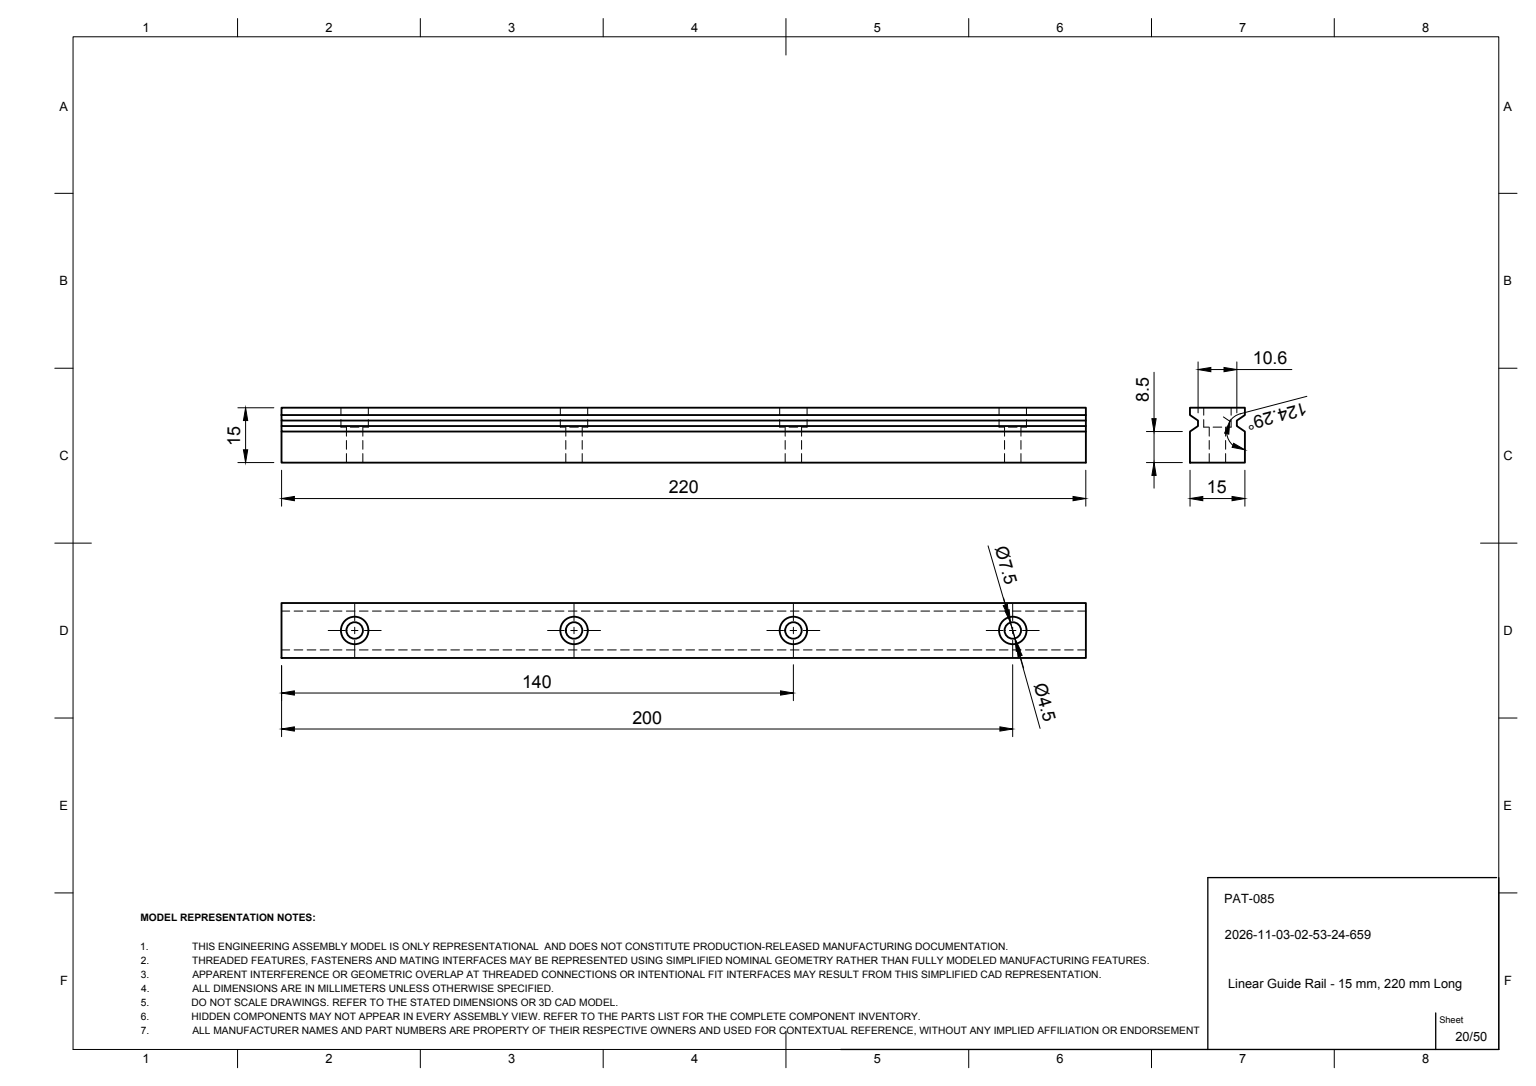
ISO-10303-21;
HEADER;
/* Generated by software containing ST-Developer
 * from STEP Tools, Inc. (www.steptools.com) 
 */

FILE_DESCRIPTION(
/* description */ ('Rack and pinion manual slide'),
/* implementation_level */ '2;1');

FILE_NAME(
/* name */ 'Linear Guide Rail - 15 mm, 220 mm Long.step',
/* time_stamp */ '2026-10-28T03:22:49-07:00',
/* author */ (''),
/* organization */ (''),
/* preprocessor_version */ 'ST-DEVELOPER v20.2',
/* originating_system */ 'Autodesk Translation Framework v15.17.0.0',
/* authorisation */ '');

FILE_SCHEMA (('AUTOMOTIVE_DESIGN { 1 0 10303 214 3 1 1 }'));
ENDSEC;

DATA;
#10=MECHANICAL_DESIGN_GEOMETRIC_PRESENTATION_REPRESENTATION('',(#749),#34851);
#657=SHAPE_REPRESENTATION_RELATIONSHIP('SRR','None',#35092,#703);
#703=ADVANCED_BREP_SHAPE_REPRESENTATION('',(#802),#34817);
#749=STYLED_ITEM('',(#35404),#802);
#802=MANIFOLD_SOLID_BREP('Body1',#13769);
#962=FACE_BOUND('',#2625,.T.);
#963=FACE_BOUND('',#2628,.T.);
#964=FACE_BOUND('',#2631,.T.);
#965=FACE_BOUND('',#2634,.T.);
#966=FACE_BOUND('',#2644,.T.);
#967=FACE_BOUND('',#2645,.T.);
#968=FACE_BOUND('',#2646,.T.);
#969=FACE_BOUND('',#2647,.T.);
#970=FACE_BOUND('',#2654,.T.);
#971=FACE_BOUND('',#2655,.T.);
#972=FACE_BOUND('',#2656,.T.);
#973=FACE_BOUND('',#2657,.T.);
#1189=PLANE('',#14713);
#1190=PLANE('',#14718);
#1191=PLANE('',#14723);
#1192=PLANE('',#14728);
#1193=PLANE('',#14738);
#1194=PLANE('',#14739);
#1195=PLANE('',#14740);
#1196=PLANE('',#14741);
#1197=PLANE('',#14742);
#1198=PLANE('',#14743);
#1199=PLANE('',#14744);
#1200=PLANE('',#14745);
#1201=PLANE('',#14746);
#1202=PLANE('',#14747);
#1203=PLANE('',#14748);
#1204=PLANE('',#14749);
#1205=PLANE('',#14750);
#1206=PLANE('',#14751);
#1755=FACE_OUTER_BOUND('',#2623,.T.);
#1756=FACE_OUTER_BOUND('',#2624,.T.);
#1757=FACE_OUTER_BOUND('',#2626,.T.);
#1758=FACE_OUTER_BOUND('',#2627,.T.);
#1759=FACE_OUTER_BOUND('',#2629,.T.);
#1760=FACE_OUTER_BOUND('',#2630,.T.);
#1761=FACE_OUTER_BOUND('',#2632,.T.);
#1762=FACE_OUTER_BOUND('',#2633,.T.);
#1763=FACE_OUTER_BOUND('',#2635,.T.);
#1764=FACE_OUTER_BOUND('',#2636,.T.);
#1765=FACE_OUTER_BOUND('',#2637,.T.);
#1766=FACE_OUTER_BOUND('',#2638,.T.);
#1767=FACE_OUTER_BOUND('',#2639,.T.);
#1768=FACE_OUTER_BOUND('',#2640,.T.);
#1769=FACE_OUTER_BOUND('',#2641,.T.);
#1770=FACE_OUTER_BOUND('',#2642,.T.);
#1771=FACE_OUTER_BOUND('',#2643,.T.);
#1772=FACE_OUTER_BOUND('',#2648,.T.);
#1773=FACE_OUTER_BOUND('',#2649,.T.);
#1774=FACE_OUTER_BOUND('',#2650,.T.);
#1775=FACE_OUTER_BOUND('',#2651,.T.);
#1776=FACE_OUTER_BOUND('',#2652,.T.);
#1777=FACE_OUTER_BOUND('',#2653,.T.);
#1778=FACE_OUTER_BOUND('',#2658,.T.);
#1779=FACE_OUTER_BOUND('',#2659,.T.);
#1780=FACE_OUTER_BOUND('',#2660,.T.);
#2623=EDGE_LOOP('',(#10306,#10307,#10308,#10309));
#2624=EDGE_LOOP('',(#10310));
#2625=EDGE_LOOP('',(#10311));
#2626=EDGE_LOOP('',(#10312,#10313,#10314,#10315));
#2627=EDGE_LOOP('',(#10316));
#2628=EDGE_LOOP('',(#10317));
#2629=EDGE_LOOP('',(#10318,#10319,#10320,#10321));
#2630=EDGE_LOOP('',(#10322));
#2631=EDGE_LOOP('',(#10323));
#2632=EDGE_LOOP('',(#10324,#10325,#10326,#10327));
#2633=EDGE_LOOP('',(#10328));
#2634=EDGE_LOOP('',(#10329));
#2635=EDGE_LOOP('',(#10330,#10331,#10332,#10333));
#2636=EDGE_LOOP('',(#10334,#10335,#10336,#10337));
#2637=EDGE_LOOP('',(#10338,#10339,#10340,#10341));
#2638=EDGE_LOOP('',(#10342,#10343,#10344,#10345));
#2639=EDGE_LOOP('',(#10346,#10347,#10348,#10349));
#2640=EDGE_LOOP('',(#10350,#10351,#10352,#10353));
#2641=EDGE_LOOP('',(#10354,#10355,#10356,#10357));
#2642=EDGE_LOOP('',(#10358,#10359,#10360,#10361));
#2643=EDGE_LOOP('',(#10362,#10363,#10364,#10365));
#2644=EDGE_LOOP('',(#10366));
#2645=EDGE_LOOP('',(#10367));
#2646=EDGE_LOOP('',(#10368));
#2647=EDGE_LOOP('',(#10369));
#2648=EDGE_LOOP('',(#10370,#10371,#10372,#10373));
#2649=EDGE_LOOP('',(#10374,#10375,#10376,#10377));
#2650=EDGE_LOOP('',(#10378,#10379,#10380,#10381));
#2651=EDGE_LOOP('',(#10382,#10383,#10384,#10385));
#2652=EDGE_LOOP('',(#10386,#10387,#10388,#10389));
#2653=EDGE_LOOP('',(#10390,#10391,#10392,#10393));
#2654=EDGE_LOOP('',(#10394));
#2655=EDGE_LOOP('',(#10395));
#2656=EDGE_LOOP('',(#10396));
#2657=EDGE_LOOP('',(#10397));
#2658=EDGE_LOOP('',(#10398,#10399,#10400,#10401));
#2659=EDGE_LOOP('',(#10402,#10403,#10404,#10405,#10406,#10407,#10408,#10409,
#10410,#10411,#10412,#10413));
#2660=EDGE_LOOP('',(#10414,#10415,#10416,#10417,#10418,#10419,#10420,#10421,
#10422,#10423,#10424,#10425));
#3607=LINE('',#20594,#4898);
#3608=LINE('',#20603,#4899);
#3609=LINE('',#20612,#4900);
#3610=LINE('',#20621,#4901);
#3611=LINE('',#20629,#4902);
#3612=LINE('',#20633,#4903);
#3613=LINE('',#20637,#4904);
#3614=LINE('',#20641,#4905);
#3615=LINE('',#20645,#4906);
#3616=LINE('',#20647,#4907);
#3617=LINE('',#20649,#4908);
#3618=LINE('',#20650,#4909);
#3619=LINE('',#20653,#4910);
#3620=LINE('',#20655,#4911);
#3621=LINE('',#20656,#4912);
#3622=LINE('',#20659,#4913);
#3623=LINE('',#20661,#4914);
#3624=LINE('',#20662,#4915);
#3625=LINE('',#20665,#4916);
#3626=LINE('',#20667,#4917);
#3627=LINE('',#20668,#4918);
#3628=LINE('',#20671,#4919);
#3629=LINE('',#20673,#4920);
#3630=LINE('',#20674,#4921);
#3631=LINE('',#20677,#4922);
#3632=LINE('',#20679,#4923);
#3633=LINE('',#20680,#4924);
#3634=LINE('',#20683,#4925);
#3635=LINE('',#20685,#4926);
#3636=LINE('',#20686,#4927);
#3637=LINE('',#20689,#4928);
#3638=LINE('',#20691,#4929);
#3639=LINE('',#20692,#4930);
#3640=LINE('',#20695,#4931);
#3641=LINE('',#20697,#4932);
#3642=LINE('',#20698,#4933);
#3643=LINE('',#20701,#4934);
#3644=LINE('',#20703,#4935);
#3645=LINE('',#20704,#4936);
#3646=LINE('',#20707,#4937);
#3647=LINE('',#20709,#4938);
#3648=LINE('',#20710,#4939);
#3649=LINE('',#20712,#4940);
#3650=LINE('',#20713,#4941);
#4898=VECTOR('',#16773,0.375);
#4899=VECTOR('',#16784,0.375);
#4900=VECTOR('',#16795,0.375);
#4901=VECTOR('',#16806,0.375);
#4902=VECTOR('',#16817,0.225);
#4903=VECTOR('',#16822,0.225);
#4904=VECTOR('',#16827,0.225);
#4905=VECTOR('',#16832,0.225000000000001);
#4906=VECTOR('',#16835,1.);
#4907=VECTOR('',#16836,1.);
#4908=VECTOR('',#16837,1.);
#4909=VECTOR('',#16838,1.);
#4910=VECTOR('',#16841,1.);
#4911=VECTOR('',#16842,1.);
#4912=VECTOR('',#16843,1.);
#4913=VECTOR('',#16846,1.);
#4914=VECTOR('',#16847,1.);
#4915=VECTOR('',#16848,1.);
#4916=VECTOR('',#16851,1.);
#4917=VECTOR('',#16852,1.);
#4918=VECTOR('',#16853,1.);
#4919=VECTOR('',#16856,1.);
#4920=VECTOR('',#16857,1.);
#4921=VECTOR('',#16858,1.);
#4922=VECTOR('',#16861,1.);
#4923=VECTOR('',#16862,1.);
#4924=VECTOR('',#16863,1.);
#4925=VECTOR('',#16866,1.);
#4926=VECTOR('',#16867,1.);
#4927=VECTOR('',#16868,1.);
#4928=VECTOR('',#16871,1.);
#4929=VECTOR('',#16872,1.);
#4930=VECTOR('',#16873,1.);
#4931=VECTOR('',#16876,1.);
#4932=VECTOR('',#16877,1.);
#4933=VECTOR('',#16878,1.);
#4934=VECTOR('',#16881,1.);
#4935=VECTOR('',#16882,1.);
#4936=VECTOR('',#16883,1.);
#4937=VECTOR('',#16886,1.);
#4938=VECTOR('',#16887,1.);
#4939=VECTOR('',#16888,1.);
#4940=VECTOR('',#16891,1.);
#4941=VECTOR('',#16892,1.);
#5957=CIRCLE('',#14711,0.375);
#5958=CIRCLE('',#14712,0.375);
#5959=CIRCLE('',#14714,0.225);
#5960=CIRCLE('',#14716,0.375);
#5961=CIRCLE('',#14717,0.375);
#5962=CIRCLE('',#14719,0.225);
#5963=CIRCLE('',#14721,0.375);
#5964=CIRCLE('',#14722,0.375);
#5965=CIRCLE('',#14724,0.225);
#5966=CIRCLE('',#14726,0.375);
#5967=CIRCLE('',#14727,0.375);
#5968=CIRCLE('',#14729,0.225000000000001);
#5969=CIRCLE('',#14731,0.225);
#5970=CIRCLE('',#14733,0.225);
#5971=CIRCLE('',#14735,0.225);
#5972=CIRCLE('',#14737,0.225000000000001);
#6581=VERTEX_POINT('',#20591);
#6582=VERTEX_POINT('',#20593);
#6583=VERTEX_POINT('',#20597);
#6584=VERTEX_POINT('',#20600);
#6585=VERTEX_POINT('',#20602);
#6586=VERTEX_POINT('',#20606);
#6587=VERTEX_POINT('',#20609);
#6588=VERTEX_POINT('',#20611);
#6589=VERTEX_POINT('',#20615);
#6590=VERTEX_POINT('',#20618);
#6591=VERTEX_POINT('',#20620);
#6592=VERTEX_POINT('',#20624);
#6593=VERTEX_POINT('',#20627);
#6594=VERTEX_POINT('',#20631);
#6595=VERTEX_POINT('',#20635);
#6596=VERTEX_POINT('',#20639);
#6597=VERTEX_POINT('',#20643);
#6598=VERTEX_POINT('',#20644);
#6599=VERTEX_POINT('',#20646);
#6600=VERTEX_POINT('',#20648);
#6601=VERTEX_POINT('',#20652);
#6602=VERTEX_POINT('',#20654);
#6603=VERTEX_POINT('',#20658);
#6604=VERTEX_POINT('',#20660);
#6605=VERTEX_POINT('',#20664);
#6606=VERTEX_POINT('',#20666);
#6607=VERTEX_POINT('',#20670);
#6608=VERTEX_POINT('',#20672);
#6609=VERTEX_POINT('',#20676);
#6610=VERTEX_POINT('',#20678);
#6611=VERTEX_POINT('',#20682);
#6612=VERTEX_POINT('',#20684);
#6613=VERTEX_POINT('',#20688);
#6614=VERTEX_POINT('',#20690);
#6615=VERTEX_POINT('',#20694);
#6616=VERTEX_POINT('',#20696);
#6617=VERTEX_POINT('',#20700);
#6618=VERTEX_POINT('',#20702);
#6619=VERTEX_POINT('',#20706);
#6620=VERTEX_POINT('',#20708);
#7965=EDGE_CURVE('',#6581,#6581,#5957,.T.);
#7966=EDGE_CURVE('',#6581,#6582,#3607,.T.);
#7967=EDGE_CURVE('',#6582,#6582,#5958,.T.);
#7968=EDGE_CURVE('',#6583,#6583,#5959,.T.);
#7969=EDGE_CURVE('',#6584,#6584,#5960,.T.);
#7970=EDGE_CURVE('',#6584,#6585,#3608,.T.);
#7971=EDGE_CURVE('',#6585,#6585,#5961,.T.);
#7972=EDGE_CURVE('',#6586,#6586,#5962,.T.);
#7973=EDGE_CURVE('',#6587,#6587,#5963,.T.);
#7974=EDGE_CURVE('',#6587,#6588,#3609,.T.);
#7975=EDGE_CURVE('',#6588,#6588,#5964,.T.);
#7976=EDGE_CURVE('',#6589,#6589,#5965,.T.);
#7977=EDGE_CURVE('',#6590,#6590,#5966,.T.);
#7978=EDGE_CURVE('',#6590,#6591,#3610,.T.);
#7979=EDGE_CURVE('',#6591,#6591,#5967,.T.);
#7980=EDGE_CURVE('',#6592,#6592,#5968,.T.);
#7981=EDGE_CURVE('',#6593,#6593,#5969,.T.);
#7982=EDGE_CURVE('',#6593,#6583,#3611,.T.);
#7983=EDGE_CURVE('',#6594,#6594,#5970,.T.);
#7984=EDGE_CURVE('',#6594,#6586,#3612,.T.);
#7985=EDGE_CURVE('',#6595,#6595,#5971,.T.);
#7986=EDGE_CURVE('',#6595,#6589,#3613,.T.);
#7987=EDGE_CURVE('',#6596,#6596,#5972,.T.);
#7988=EDGE_CURVE('',#6596,#6592,#3614,.T.);
#7989=EDGE_CURVE('',#6597,#6598,#3615,.T.);
#7990=EDGE_CURVE('',#6598,#6599,#3616,.T.);
#7991=EDGE_CURVE('',#6600,#6599,#3617,.T.);
#7992=EDGE_CURVE('',#6597,#6600,#3618,.T.);
#7993=EDGE_CURVE('',#6601,#6597,#3619,.T.);
#7994=EDGE_CURVE('',#6602,#6600,#3620,.T.);
#7995=EDGE_CURVE('',#6601,#6602,#3621,.T.);
#7996=EDGE_CURVE('',#6603,#6601,#3622,.T.);
#7997=EDGE_CURVE('',#6604,#6602,#3623,.T.);
#7998=EDGE_CURVE('',#6603,#6604,#3624,.T.);
#7999=EDGE_CURVE('',#6605,#6603,#3625,.T.);
#8000=EDGE_CURVE('',#6606,#6604,#3626,.T.);
#8001=EDGE_CURVE('',#6605,#6606,#3627,.T.);
#8002=EDGE_CURVE('',#6607,#6605,#3628,.T.);
#8003=EDGE_CURVE('',#6608,#6606,#3629,.T.);
#8004=EDGE_CURVE('',#6607,#6608,#3630,.T.);
#8005=EDGE_CURVE('',#6609,#6607,#3631,.T.);
#8006=EDGE_CURVE('',#6610,#6608,#3632,.T.);
#8007=EDGE_CURVE('',#6609,#6610,#3633,.T.);
#8008=EDGE_CURVE('',#6611,#6609,#3634,.T.);
#8009=EDGE_CURVE('',#6612,#6610,#3635,.T.);
#8010=EDGE_CURVE('',#6611,#6612,#3636,.T.);
#8011=EDGE_CURVE('',#6613,#6611,#3637,.T.);
#8012=EDGE_CURVE('',#6614,#6612,#3638,.T.);
#8013=EDGE_CURVE('',#6613,#6614,#3639,.T.);
#8014=EDGE_CURVE('',#6615,#6613,#3640,.T.);
#8015=EDGE_CURVE('',#6616,#6614,#3641,.T.);
#8016=EDGE_CURVE('',#6615,#6616,#3642,.T.);
#8017=EDGE_CURVE('',#6617,#6615,#3643,.T.);
#8018=EDGE_CURVE('',#6618,#6616,#3644,.T.);
#8019=EDGE_CURVE('',#6617,#6618,#3645,.T.);
#8020=EDGE_CURVE('',#6619,#6617,#3646,.T.);
#8021=EDGE_CURVE('',#6620,#6618,#3647,.T.);
#8022=EDGE_CURVE('',#6619,#6620,#3648,.T.);
#8023=EDGE_CURVE('',#6598,#6619,#3649,.T.);
#8024=EDGE_CURVE('',#6599,#6620,#3650,.T.);
#10306=ORIENTED_EDGE('',*,*,#7965,.F.);
#10307=ORIENTED_EDGE('',*,*,#7966,.T.);
#10308=ORIENTED_EDGE('',*,*,#7967,.F.);
#10309=ORIENTED_EDGE('',*,*,#7966,.F.);
#10310=ORIENTED_EDGE('',*,*,#7965,.T.);
#10311=ORIENTED_EDGE('',*,*,#7968,.F.);
#10312=ORIENTED_EDGE('',*,*,#7969,.F.);
#10313=ORIENTED_EDGE('',*,*,#7970,.T.);
#10314=ORIENTED_EDGE('',*,*,#7971,.F.);
#10315=ORIENTED_EDGE('',*,*,#7970,.F.);
#10316=ORIENTED_EDGE('',*,*,#7969,.T.);
#10317=ORIENTED_EDGE('',*,*,#7972,.F.);
#10318=ORIENTED_EDGE('',*,*,#7973,.F.);
#10319=ORIENTED_EDGE('',*,*,#7974,.T.);
#10320=ORIENTED_EDGE('',*,*,#7975,.F.);
#10321=ORIENTED_EDGE('',*,*,#7974,.F.);
#10322=ORIENTED_EDGE('',*,*,#7973,.T.);
#10323=ORIENTED_EDGE('',*,*,#7976,.F.);
#10324=ORIENTED_EDGE('',*,*,#7977,.F.);
#10325=ORIENTED_EDGE('',*,*,#7978,.T.);
#10326=ORIENTED_EDGE('',*,*,#7979,.F.);
#10327=ORIENTED_EDGE('',*,*,#7978,.F.);
#10328=ORIENTED_EDGE('',*,*,#7977,.T.);
#10329=ORIENTED_EDGE('',*,*,#7980,.F.);
#10330=ORIENTED_EDGE('',*,*,#7981,.F.);
#10331=ORIENTED_EDGE('',*,*,#7982,.T.);
#10332=ORIENTED_EDGE('',*,*,#7968,.T.);
#10333=ORIENTED_EDGE('',*,*,#7982,.F.);
#10334=ORIENTED_EDGE('',*,*,#7983,.F.);
#10335=ORIENTED_EDGE('',*,*,#7984,.T.);
#10336=ORIENTED_EDGE('',*,*,#7972,.T.);
#10337=ORIENTED_EDGE('',*,*,#7984,.F.);
#10338=ORIENTED_EDGE('',*,*,#7985,.F.);
#10339=ORIENTED_EDGE('',*,*,#7986,.T.);
#10340=ORIENTED_EDGE('',*,*,#7976,.T.);
#10341=ORIENTED_EDGE('',*,*,#7986,.F.);
#10342=ORIENTED_EDGE('',*,*,#7987,.F.);
#10343=ORIENTED_EDGE('',*,*,#7988,.T.);
#10344=ORIENTED_EDGE('',*,*,#7980,.T.);
#10345=ORIENTED_EDGE('',*,*,#7988,.F.);
#10346=ORIENTED_EDGE('',*,*,#7989,.T.);
#10347=ORIENTED_EDGE('',*,*,#7990,.T.);
#10348=ORIENTED_EDGE('',*,*,#7991,.F.);
#10349=ORIENTED_EDGE('',*,*,#7992,.F.);
#10350=ORIENTED_EDGE('',*,*,#7993,.T.);
#10351=ORIENTED_EDGE('',*,*,#7992,.T.);
#10352=ORIENTED_EDGE('',*,*,#7994,.F.);
#10353=ORIENTED_EDGE('',*,*,#7995,.F.);
#10354=ORIENTED_EDGE('',*,*,#7996,.T.);
#10355=ORIENTED_EDGE('',*,*,#7995,.T.);
#10356=ORIENTED_EDGE('',*,*,#7997,.F.);
#10357=ORIENTED_EDGE('',*,*,#7998,.F.);
#10358=ORIENTED_EDGE('',*,*,#7999,.T.);
#10359=ORIENTED_EDGE('',*,*,#7998,.T.);
#10360=ORIENTED_EDGE('',*,*,#8000,.F.);
#10361=ORIENTED_EDGE('',*,*,#8001,.F.);
#10362=ORIENTED_EDGE('',*,*,#8002,.T.);
#10363=ORIENTED_EDGE('',*,*,#8001,.T.);
#10364=ORIENTED_EDGE('',*,*,#8003,.F.);
#10365=ORIENTED_EDGE('',*,*,#8004,.F.);
#10366=ORIENTED_EDGE('',*,*,#7979,.T.);
#10367=ORIENTED_EDGE('',*,*,#7975,.T.);
#10368=ORIENTED_EDGE('',*,*,#7971,.T.);
#10369=ORIENTED_EDGE('',*,*,#7967,.T.);
#10370=ORIENTED_EDGE('',*,*,#8005,.T.);
#10371=ORIENTED_EDGE('',*,*,#8004,.T.);
#10372=ORIENTED_EDGE('',*,*,#8006,.F.);
#10373=ORIENTED_EDGE('',*,*,#8007,.F.);
#10374=ORIENTED_EDGE('',*,*,#8008,.T.);
#10375=ORIENTED_EDGE('',*,*,#8007,.T.);
#10376=ORIENTED_EDGE('',*,*,#8009,.F.);
#10377=ORIENTED_EDGE('',*,*,#8010,.F.);
#10378=ORIENTED_EDGE('',*,*,#8011,.T.);
#10379=ORIENTED_EDGE('',*,*,#8010,.T.);
#10380=ORIENTED_EDGE('',*,*,#8012,.F.);
#10381=ORIENTED_EDGE('',*,*,#8013,.F.);
#10382=ORIENTED_EDGE('',*,*,#8014,.T.);
#10383=ORIENTED_EDGE('',*,*,#8013,.T.);
#10384=ORIENTED_EDGE('',*,*,#8015,.F.);
#10385=ORIENTED_EDGE('',*,*,#8016,.F.);
#10386=ORIENTED_EDGE('',*,*,#8017,.T.);
#10387=ORIENTED_EDGE('',*,*,#8016,.T.);
#10388=ORIENTED_EDGE('',*,*,#8018,.F.);
#10389=ORIENTED_EDGE('',*,*,#8019,.F.);
#10390=ORIENTED_EDGE('',*,*,#8020,.T.);
#10391=ORIENTED_EDGE('',*,*,#8019,.T.);
#10392=ORIENTED_EDGE('',*,*,#8021,.F.);
#10393=ORIENTED_EDGE('',*,*,#8022,.F.);
#10394=ORIENTED_EDGE('',*,*,#7981,.T.);
#10395=ORIENTED_EDGE('',*,*,#7983,.T.);
#10396=ORIENTED_EDGE('',*,*,#7985,.T.);
#10397=ORIENTED_EDGE('',*,*,#7987,.T.);
#10398=ORIENTED_EDGE('',*,*,#8023,.T.);
#10399=ORIENTED_EDGE('',*,*,#8022,.T.);
#10400=ORIENTED_EDGE('',*,*,#8024,.F.);
#10401=ORIENTED_EDGE('',*,*,#7990,.F.);
#10402=ORIENTED_EDGE('',*,*,#8024,.T.);
#10403=ORIENTED_EDGE('',*,*,#8021,.T.);
#10404=ORIENTED_EDGE('',*,*,#8018,.T.);
#10405=ORIENTED_EDGE('',*,*,#8015,.T.);
#10406=ORIENTED_EDGE('',*,*,#8012,.T.);
#10407=ORIENTED_EDGE('',*,*,#8009,.T.);
#10408=ORIENTED_EDGE('',*,*,#8006,.T.);
#10409=ORIENTED_EDGE('',*,*,#8003,.T.);
#10410=ORIENTED_EDGE('',*,*,#8000,.T.);
#10411=ORIENTED_EDGE('',*,*,#7997,.T.);
#10412=ORIENTED_EDGE('',*,*,#7994,.T.);
#10413=ORIENTED_EDGE('',*,*,#7991,.T.);
#10414=ORIENTED_EDGE('',*,*,#8023,.F.);
#10415=ORIENTED_EDGE('',*,*,#7989,.F.);
#10416=ORIENTED_EDGE('',*,*,#7993,.F.);
#10417=ORIENTED_EDGE('',*,*,#7996,.F.);
#10418=ORIENTED_EDGE('',*,*,#7999,.F.);
#10419=ORIENTED_EDGE('',*,*,#8002,.F.);
#10420=ORIENTED_EDGE('',*,*,#8005,.F.);
#10421=ORIENTED_EDGE('',*,*,#8008,.F.);
#10422=ORIENTED_EDGE('',*,*,#8011,.F.);
#10423=ORIENTED_EDGE('',*,*,#8014,.F.);
#10424=ORIENTED_EDGE('',*,*,#8017,.F.);
#10425=ORIENTED_EDGE('',*,*,#8020,.F.);
#12918=CYLINDRICAL_SURFACE('',#14710,0.375);
#12919=CYLINDRICAL_SURFACE('',#14715,0.375);
#12920=CYLINDRICAL_SURFACE('',#14720,0.375);
#12921=CYLINDRICAL_SURFACE('',#14725,0.375);
#12922=CYLINDRICAL_SURFACE('',#14730,0.225);
#12923=CYLINDRICAL_SURFACE('',#14732,0.225);
#12924=CYLINDRICAL_SURFACE('',#14734,0.225);
#12925=CYLINDRICAL_SURFACE('',#14736,0.225000000000001);
#13233=ADVANCED_FACE('',(#1755),#12918,.F.);
#13234=ADVANCED_FACE('',(#1756,#962),#1189,.T.);
#13235=ADVANCED_FACE('',(#1757),#12919,.F.);
#13236=ADVANCED_FACE('',(#1758,#963),#1190,.T.);
#13237=ADVANCED_FACE('',(#1759),#12920,.F.);
#13238=ADVANCED_FACE('',(#1760,#964),#1191,.T.);
#13239=ADVANCED_FACE('',(#1761),#12921,.F.);
#13240=ADVANCED_FACE('',(#1762,#965),#1192,.T.);
#13241=ADVANCED_FACE('',(#1763),#12922,.F.);
#13242=ADVANCED_FACE('',(#1764),#12923,.F.);
#13243=ADVANCED_FACE('',(#1765),#12924,.F.);
#13244=ADVANCED_FACE('',(#1766),#12925,.F.);
#13245=ADVANCED_FACE('',(#1767),#1193,.T.);
#13246=ADVANCED_FACE('',(#1768),#1194,.T.);
#13247=ADVANCED_FACE('',(#1769),#1195,.T.);
#13248=ADVANCED_FACE('',(#1770),#1196,.T.);
#13249=ADVANCED_FACE('',(#1771,#966,#967,#968,#969),#1197,.T.);
#13250=ADVANCED_FACE('',(#1772),#1198,.T.);
#13251=ADVANCED_FACE('',(#1773),#1199,.T.);
#13252=ADVANCED_FACE('',(#1774),#1200,.T.);
#13253=ADVANCED_FACE('',(#1775),#1201,.T.);
#13254=ADVANCED_FACE('',(#1776),#1202,.T.);
#13255=ADVANCED_FACE('',(#1777,#970,#971,#972,#973),#1203,.T.);
#13256=ADVANCED_FACE('',(#1778),#1204,.T.);
#13257=ADVANCED_FACE('',(#1779),#1205,.T.);
#13258=ADVANCED_FACE('',(#1780),#1206,.F.);
#13769=CLOSED_SHELL('',(#13233,#13234,#13235,#13236,#13237,#13238,#13239,
#13240,#13241,#13242,#13243,#13244,#13245,#13246,#13247,#13248,#13249,#13250,
#13251,#13252,#13253,#13254,#13255,#13256,#13257,#13258));
#14709=AXIS2_PLACEMENT_3D('',#20589,#16767,#16768);
#14710=AXIS2_PLACEMENT_3D('',#20590,#16769,#16770);
#14711=AXIS2_PLACEMENT_3D('',#20592,#16771,#16772);
#14712=AXIS2_PLACEMENT_3D('',#20595,#16774,#16775);
#14713=AXIS2_PLACEMENT_3D('',#20596,#16776,#16777);
#14714=AXIS2_PLACEMENT_3D('',#20598,#16778,#16779);
#14715=AXIS2_PLACEMENT_3D('',#20599,#16780,#16781);
#14716=AXIS2_PLACEMENT_3D('',#20601,#16782,#16783);
#14717=AXIS2_PLACEMENT_3D('',#20604,#16785,#16786);
#14718=AXIS2_PLACEMENT_3D('',#20605,#16787,#16788);
#14719=AXIS2_PLACEMENT_3D('',#20607,#16789,#16790);
#14720=AXIS2_PLACEMENT_3D('',#20608,#16791,#16792);
#14721=AXIS2_PLACEMENT_3D('',#20610,#16793,#16794);
#14722=AXIS2_PLACEMENT_3D('',#20613,#16796,#16797);
#14723=AXIS2_PLACEMENT_3D('',#20614,#16798,#16799);
#14724=AXIS2_PLACEMENT_3D('',#20616,#16800,#16801);
#14725=AXIS2_PLACEMENT_3D('',#20617,#16802,#16803);
#14726=AXIS2_PLACEMENT_3D('',#20619,#16804,#16805);
#14727=AXIS2_PLACEMENT_3D('',#20622,#16807,#16808);
#14728=AXIS2_PLACEMENT_3D('',#20623,#16809,#16810);
#14729=AXIS2_PLACEMENT_3D('',#20625,#16811,#16812);
#14730=AXIS2_PLACEMENT_3D('',#20626,#16813,#16814);
#14731=AXIS2_PLACEMENT_3D('',#20628,#16815,#16816);
#14732=AXIS2_PLACEMENT_3D('',#20630,#16818,#16819);
#14733=AXIS2_PLACEMENT_3D('',#20632,#16820,#16821);
#14734=AXIS2_PLACEMENT_3D('',#20634,#16823,#16824);
#14735=AXIS2_PLACEMENT_3D('',#20636,#16825,#16826);
#14736=AXIS2_PLACEMENT_3D('',#20638,#16828,#16829);
#14737=AXIS2_PLACEMENT_3D('',#20640,#16830,#16831);
#14738=AXIS2_PLACEMENT_3D('',#20642,#16833,#16834);
#14739=AXIS2_PLACEMENT_3D('',#20651,#16839,#16840);
#14740=AXIS2_PLACEMENT_3D('',#20657,#16844,#16845);
#14741=AXIS2_PLACEMENT_3D('',#20663,#16849,#16850);
#14742=AXIS2_PLACEMENT_3D('',#20669,#16854,#16855);
#14743=AXIS2_PLACEMENT_3D('',#20675,#16859,#16860);
#14744=AXIS2_PLACEMENT_3D('',#20681,#16864,#16865);
#14745=AXIS2_PLACEMENT_3D('',#20687,#16869,#16870);
#14746=AXIS2_PLACEMENT_3D('',#20693,#16874,#16875);
#14747=AXIS2_PLACEMENT_3D('',#20699,#16879,#16880);
#14748=AXIS2_PLACEMENT_3D('',#20705,#16884,#16885);
#14749=AXIS2_PLACEMENT_3D('',#20711,#16889,#16890);
#14750=AXIS2_PLACEMENT_3D('',#20714,#16893,#16894);
#14751=AXIS2_PLACEMENT_3D('',#20715,#16895,#16896);
#16767=DIRECTION('axis',(0.,0.,1.));
#16768=DIRECTION('refdir',(1.,0.,0.));
#16769=DIRECTION('center_axis',(0.,0.,1.));
#16770=DIRECTION('ref_axis',(1.,0.,0.));
#16771=DIRECTION('center_axis',(0.,0.,1.));
#16772=DIRECTION('ref_axis',(1.,0.,0.));
#16773=DIRECTION('',(0.,0.,1.));
#16774=DIRECTION('center_axis',(0.,0.,-1.));
#16775=DIRECTION('ref_axis',(1.,0.,0.));
#16776=DIRECTION('center_axis',(0.,0.,1.));
#16777=DIRECTION('ref_axis',(1.,0.,0.));
#16778=DIRECTION('center_axis',(0.,0.,1.));
#16779=DIRECTION('ref_axis',(1.,0.,0.));
#16780=DIRECTION('center_axis',(0.,0.,1.));
#16781=DIRECTION('ref_axis',(1.,0.,0.));
#16782=DIRECTION('center_axis',(0.,0.,1.));
#16783=DIRECTION('ref_axis',(1.,0.,0.));
#16784=DIRECTION('',(0.,0.,1.));
#16785=DIRECTION('center_axis',(0.,0.,-1.));
#16786=DIRECTION('ref_axis',(1.,0.,0.));
#16787=DIRECTION('center_axis',(0.,0.,1.));
#16788=DIRECTION('ref_axis',(1.,0.,0.));
#16789=DIRECTION('center_axis',(0.,0.,1.));
#16790=DIRECTION('ref_axis',(1.,0.,0.));
#16791=DIRECTION('center_axis',(0.,0.,1.));
#16792=DIRECTION('ref_axis',(1.,0.,0.));
#16793=DIRECTION('center_axis',(0.,0.,1.));
#16794=DIRECTION('ref_axis',(1.,0.,0.));
#16795=DIRECTION('',(0.,0.,1.));
#16796=DIRECTION('center_axis',(0.,0.,-1.));
#16797=DIRECTION('ref_axis',(1.,0.,0.));
#16798=DIRECTION('center_axis',(0.,0.,1.));
#16799=DIRECTION('ref_axis',(1.,0.,0.));
#16800=DIRECTION('center_axis',(0.,0.,1.));
#16801=DIRECTION('ref_axis',(1.,0.,0.));
#16802=DIRECTION('center_axis',(0.,0.,1.));
#16803=DIRECTION('ref_axis',(1.,0.,0.));
#16804=DIRECTION('center_axis',(0.,0.,1.));
#16805=DIRECTION('ref_axis',(1.,0.,0.));
#16806=DIRECTION('',(0.,0.,1.));
#16807=DIRECTION('center_axis',(0.,0.,-1.));
#16808=DIRECTION('ref_axis',(1.,0.,0.));
#16809=DIRECTION('center_axis',(0.,0.,1.));
#16810=DIRECTION('ref_axis',(1.,0.,0.));
#16811=DIRECTION('center_axis',(0.,0.,1.));
#16812=DIRECTION('ref_axis',(1.,0.,0.));
#16813=DIRECTION('center_axis',(0.,0.,1.));
#16814=DIRECTION('ref_axis',(1.,0.,0.));
#16815=DIRECTION('center_axis',(0.,0.,1.));
#16816=DIRECTION('ref_axis',(1.,0.,0.));
#16817=DIRECTION('',(0.,0.,1.));
#16818=DIRECTION('center_axis',(0.,0.,1.));
#16819=DIRECTION('ref_axis',(1.,0.,0.));
#16820=DIRECTION('center_axis',(0.,0.,1.));
#16821=DIRECTION('ref_axis',(1.,0.,0.));
#16822=DIRECTION('',(0.,0.,1.));
#16823=DIRECTION('center_axis',(0.,0.,1.));
#16824=DIRECTION('ref_axis',(1.,0.,0.));
#16825=DIRECTION('center_axis',(0.,0.,1.));
#16826=DIRECTION('ref_axis',(1.,0.,0.));
#16827=DIRECTION('',(0.,0.,1.));
#16828=DIRECTION('center_axis',(0.,0.,1.));
#16829=DIRECTION('ref_axis',(1.,0.,0.));
#16830=DIRECTION('center_axis',(0.,0.,1.));
#16831=DIRECTION('ref_axis',(1.,0.,0.));
#16832=DIRECTION('',(0.,0.,1.));
#16833=DIRECTION('center_axis',(0.,-0.56333682464151,0.826227342807548));
#16834=DIRECTION('ref_axis',(0.,-0.826227342807548,-0.56333682464151));
#16835=DIRECTION('',(0.,-0.826227342807548,-0.56333682464151));
#16836=DIRECTION('',(1.,0.,0.));
#16837=DIRECTION('',(0.,-0.826227342807548,-0.56333682464151));
#16838=DIRECTION('',(1.,0.,0.));
#16839=DIRECTION('center_axis',(0.,-1.,0.));
#16840=DIRECTION('ref_axis',(0.,0.,-1.));
#16841=DIRECTION('',(0.,0.,-1.));
#16842=DIRECTION('',(0.,0.,-1.));
#16843=DIRECTION('',(1.,0.,0.));
#16844=DIRECTION('center_axis',(0.,-0.56333682464151,-0.826227342807548));
#16845=DIRECTION('ref_axis',(0.,0.826227342807548,-0.56333682464151));
#16846=DIRECTION('',(0.,0.826227342807548,-0.56333682464151));
#16847=DIRECTION('',(0.,0.826227342807548,-0.56333682464151));
#16848=DIRECTION('',(1.,0.,0.));
#16849=DIRECTION('center_axis',(0.,-1.,0.));
#16850=DIRECTION('ref_axis',(0.,0.,-1.));
#16851=DIRECTION('',(0.,0.,-1.));
#16852=DIRECTION('',(0.,0.,-1.));
#16853=DIRECTION('',(1.,0.,0.));
#16854=DIRECTION('center_axis',(0.,0.,1.));
#16855=DIRECTION('ref_axis',(0.,-1.,0.));
#16856=DIRECTION('',(0.,-1.,0.));
#16857=DIRECTION('',(0.,-1.,0.));
#16858=DIRECTION('',(1.,0.,0.));
#16859=DIRECTION('center_axis',(0.,1.,0.));
#16860=DIRECTION('ref_axis',(0.,0.,1.));
#16861=DIRECTION('',(0.,0.,1.));
#16862=DIRECTION('',(0.,0.,1.));
#16863=DIRECTION('',(1.,0.,0.));
#16864=DIRECTION('center_axis',(0.,0.56333682464151,-0.826227342807548));
#16865=DIRECTION('ref_axis',(0.,0.826227342807548,0.56333682464151));
#16866=DIRECTION('',(0.,0.826227342807548,0.56333682464151));
#16867=DIRECTION('',(0.,0.826227342807548,0.56333682464151));
#16868=DIRECTION('',(1.,0.,0.));
#16869=DIRECTION('center_axis',(0.,1.,0.));
#16870=DIRECTION('ref_axis',(0.,0.,1.));
#16871=DIRECTION('',(0.,0.,1.));
#16872=DIRECTION('',(0.,0.,1.));
#16873=DIRECTION('',(1.,0.,0.));
#16874=DIRECTION('center_axis',(0.,0.56333682464151,0.826227342807548));
#16875=DIRECTION('ref_axis',(0.,-0.826227342807548,0.56333682464151));
#16876=DIRECTION('',(0.,-0.826227342807548,0.56333682464151));
#16877=DIRECTION('',(0.,-0.826227342807548,0.56333682464151));
#16878=DIRECTION('',(1.,0.,0.));
#16879=DIRECTION('center_axis',(0.,1.,0.));
#16880=DIRECTION('ref_axis',(0.,0.,1.));
#16881=DIRECTION('',(0.,0.,1.));
#16882=DIRECTION('',(0.,0.,1.));
#16883=DIRECTION('',(1.,0.,0.));
#16884=DIRECTION('center_axis',(0.,0.,-1.));
#16885=DIRECTION('ref_axis',(0.,1.,0.));
#16886=DIRECTION('',(0.,1.,0.));
#16887=DIRECTION('',(0.,1.,0.));
#16888=DIRECTION('',(1.,0.,0.));
#16889=DIRECTION('center_axis',(0.,-1.,0.));
#16890=DIRECTION('ref_axis',(0.,0.,-1.));
#16891=DIRECTION('',(0.,0.,-1.));
#16892=DIRECTION('',(0.,0.,-1.));
#16893=DIRECTION('center_axis',(1.,0.,0.));
#16894=DIRECTION('ref_axis',(0.,0.,-1.));
#16895=DIRECTION('center_axis',(1.,0.,0.));
#16896=DIRECTION('ref_axis',(0.,0.,-1.));
#20589=CARTESIAN_POINT('',(0.,0.,0.));
#20590=CARTESIAN_POINT('Origin',(14.,0.,0.97));
#20591=CARTESIAN_POINT('',(13.625,-4.59242549680257E-17,0.97));
#20592=CARTESIAN_POINT('Origin',(14.,0.,0.97));
#20593=CARTESIAN_POINT('',(13.625,4.59242549680257E-17,1.5));
#20594=CARTESIAN_POINT('',(13.625,-4.59242549680257E-17,0.97));
#20595=CARTESIAN_POINT('Origin',(14.,0.,1.5));
#20596=CARTESIAN_POINT('Origin',(14.,0.,0.97));
#20597=CARTESIAN_POINT('',(13.775,-2.75545529808154E-17,0.97));
#20598=CARTESIAN_POINT('Origin',(14.,0.,0.97));
#20599=CARTESIAN_POINT('Origin',(8.,0.,0.97));
#20600=CARTESIAN_POINT('',(7.625,-4.59242549680257E-17,0.97));
#20601=CARTESIAN_POINT('Origin',(8.,0.,0.97));
#20602=CARTESIAN_POINT('',(7.625,4.59242549680257E-17,1.5));
#20603=CARTESIAN_POINT('',(7.625,-4.59242549680257E-17,0.97));
#20604=CARTESIAN_POINT('Origin',(8.,0.,1.5));
#20605=CARTESIAN_POINT('Origin',(8.,0.,0.97));
#20606=CARTESIAN_POINT('',(7.775,-2.75545529808154E-17,0.97));
#20607=CARTESIAN_POINT('Origin',(8.,0.,0.97));
#20608=CARTESIAN_POINT('Origin',(2.,0.,0.97));
#20609=CARTESIAN_POINT('',(1.625,-4.59242549680257E-17,0.97));
#20610=CARTESIAN_POINT('Origin',(2.,0.,0.97));
#20611=CARTESIAN_POINT('',(1.625,4.59242549680257E-17,1.5));
#20612=CARTESIAN_POINT('',(1.625,-4.59242549680257E-17,0.97));
#20613=CARTESIAN_POINT('Origin',(2.,0.,1.5));
#20614=CARTESIAN_POINT('Origin',(2.,0.,0.97));
#20615=CARTESIAN_POINT('',(1.775,-2.75545529808155E-17,0.97));
#20616=CARTESIAN_POINT('Origin',(2.,0.,0.97));
#20617=CARTESIAN_POINT('Origin',(20.,0.,0.97));
#20618=CARTESIAN_POINT('',(19.625,-4.59242549680257E-17,0.97));
#20619=CARTESIAN_POINT('Origin',(20.,0.,0.97));
#20620=CARTESIAN_POINT('',(19.625,4.59242549680257E-17,1.5));
#20621=CARTESIAN_POINT('',(19.625,-4.59242549680257E-17,0.97));
#20622=CARTESIAN_POINT('Origin',(20.,0.,1.5));
#20623=CARTESIAN_POINT('Origin',(20.,0.,0.97));
#20624=CARTESIAN_POINT('',(19.775,-2.75545529808156E-17,0.97));
#20625=CARTESIAN_POINT('Origin',(20.,0.,0.97));
#20626=CARTESIAN_POINT('Origin',(14.,0.,-0.1));
#20627=CARTESIAN_POINT('',(13.775,-2.75545529808154E-17,0.));
#20628=CARTESIAN_POINT('Origin',(14.,0.,0.));
#20629=CARTESIAN_POINT('',(13.775,-2.75545529808154E-17,-0.1));
#20630=CARTESIAN_POINT('Origin',(8.,0.,-0.1));
#20631=CARTESIAN_POINT('',(7.775,-2.75545529808154E-17,0.));
#20632=CARTESIAN_POINT('Origin',(8.,0.,0.));
#20633=CARTESIAN_POINT('',(7.775,-2.75545529808154E-17,-0.1));
#20634=CARTESIAN_POINT('Origin',(2.,0.,-0.1));
#20635=CARTESIAN_POINT('',(1.775,-2.75545529808155E-17,0.));
#20636=CARTESIAN_POINT('Origin',(2.,0.,0.));
#20637=CARTESIAN_POINT('',(1.775,-2.75545529808155E-17,-0.1));
#20638=CARTESIAN_POINT('Origin',(20.,0.,-0.1));
#20639=CARTESIAN_POINT('',(19.775,-2.75545529808156E-17,0.));
#20640=CARTESIAN_POINT('Origin',(20.,0.,0.));
#20641=CARTESIAN_POINT('',(19.775,-2.75545529808156E-17,-0.1));
#20642=CARTESIAN_POINT('Origin',(0.,-0.53,1.));
#20643=CARTESIAN_POINT('',(0.,-0.53,1.));
#20644=CARTESIAN_POINT('',(0.,-0.75,0.85));
#20645=CARTESIAN_POINT('',(0.,-0.53,1.));
#20646=CARTESIAN_POINT('',(22.,-0.75,0.85));
#20647=CARTESIAN_POINT('',(0.,-0.75,0.85));
#20648=CARTESIAN_POINT('',(22.,-0.53,1.));
#20649=CARTESIAN_POINT('',(22.,-0.53,1.));
#20650=CARTESIAN_POINT('',(0.,-0.53,1.));
#20651=CARTESIAN_POINT('Origin',(0.,-0.53,1.15));
#20652=CARTESIAN_POINT('',(0.,-0.53,1.15));
#20653=CARTESIAN_POINT('',(0.,-0.53,1.15));
#20654=CARTESIAN_POINT('',(22.,-0.53,1.15));
#20655=CARTESIAN_POINT('',(22.,-0.53,1.15));
#20656=CARTESIAN_POINT('',(0.,-0.53,1.15));
#20657=CARTESIAN_POINT('Origin',(0.,-0.75,1.3));
#20658=CARTESIAN_POINT('',(0.,-0.75,1.3));
#20659=CARTESIAN_POINT('',(0.,-0.75,1.3));
#20660=CARTESIAN_POINT('',(22.,-0.75,1.3));
#20661=CARTESIAN_POINT('',(22.,-0.75,1.3));
#20662=CARTESIAN_POINT('',(0.,-0.75,1.3));
#20663=CARTESIAN_POINT('Origin',(0.,-0.75,1.5));
#20664=CARTESIAN_POINT('',(0.,-0.75,1.5));
#20665=CARTESIAN_POINT('',(0.,-0.75,1.5));
#20666=CARTESIAN_POINT('',(22.,-0.75,1.5));
#20667=CARTESIAN_POINT('',(22.,-0.75,1.5));
#20668=CARTESIAN_POINT('',(0.,-0.75,1.5));
#20669=CARTESIAN_POINT('Origin',(0.,0.75,1.5));
#20670=CARTESIAN_POINT('',(0.,0.75,1.5));
#20671=CARTESIAN_POINT('',(0.,0.75,1.5));
#20672=CARTESIAN_POINT('',(22.,0.75,1.5));
#20673=CARTESIAN_POINT('',(22.,0.75,1.5));
#20674=CARTESIAN_POINT('',(0.,0.75,1.5));
#20675=CARTESIAN_POINT('Origin',(0.,0.75,1.3));
#20676=CARTESIAN_POINT('',(0.,0.75,1.3));
#20677=CARTESIAN_POINT('',(0.,0.75,1.3));
#20678=CARTESIAN_POINT('',(22.,0.75,1.3));
#20679=CARTESIAN_POINT('',(22.,0.75,1.3));
#20680=CARTESIAN_POINT('',(0.,0.75,1.3));
#20681=CARTESIAN_POINT('Origin',(0.,0.53,1.15));
#20682=CARTESIAN_POINT('',(0.,0.53,1.15));
#20683=CARTESIAN_POINT('',(0.,0.53,1.15));
#20684=CARTESIAN_POINT('',(22.,0.53,1.15));
#20685=CARTESIAN_POINT('',(22.,0.53,1.15));
#20686=CARTESIAN_POINT('',(0.,0.53,1.15));
#20687=CARTESIAN_POINT('Origin',(0.,0.53,1.));
#20688=CARTESIAN_POINT('',(0.,0.53,1.));
#20689=CARTESIAN_POINT('',(0.,0.53,1.));
#20690=CARTESIAN_POINT('',(22.,0.53,1.));
#20691=CARTESIAN_POINT('',(22.,0.53,1.));
#20692=CARTESIAN_POINT('',(0.,0.53,1.));
#20693=CARTESIAN_POINT('Origin',(0.,0.75,0.85));
#20694=CARTESIAN_POINT('',(0.,0.75,0.85));
#20695=CARTESIAN_POINT('',(0.,0.75,0.85));
#20696=CARTESIAN_POINT('',(22.,0.75,0.85));
#20697=CARTESIAN_POINT('',(22.,0.75,0.85));
#20698=CARTESIAN_POINT('',(0.,0.75,0.85));
#20699=CARTESIAN_POINT('Origin',(0.,0.75,0.));
#20700=CARTESIAN_POINT('',(0.,0.75,0.));
#20701=CARTESIAN_POINT('',(0.,0.75,0.));
#20702=CARTESIAN_POINT('',(22.,0.75,0.));
#20703=CARTESIAN_POINT('',(22.,0.75,0.));
#20704=CARTESIAN_POINT('',(0.,0.75,0.));
#20705=CARTESIAN_POINT('Origin',(0.,-0.75,0.));
#20706=CARTESIAN_POINT('',(0.,-0.75,0.));
#20707=CARTESIAN_POINT('',(0.,-0.75,0.));
#20708=CARTESIAN_POINT('',(22.,-0.75,0.));
#20709=CARTESIAN_POINT('',(22.,-0.75,0.));
#20710=CARTESIAN_POINT('',(0.,-0.75,0.));
#20711=CARTESIAN_POINT('Origin',(0.,-0.75,0.85));
#20712=CARTESIAN_POINT('',(0.,-0.75,0.85));
#20713=CARTESIAN_POINT('',(22.,-0.75,0.85));
#20714=CARTESIAN_POINT('Origin',(22.,0.,0.75));
#20715=CARTESIAN_POINT('Origin',(0.,0.,0.75));
#34763=UNCERTAINTY_MEASURE_WITH_UNIT(LENGTH_MEASURE(0.001),#34852,
'DISTANCE_ACCURACY_VALUE',
'Maximum model space distance between geometric entities at asserted c
onnectivities');
#34797=UNCERTAINTY_MEASURE_WITH_UNIT(LENGTH_MEASURE(0.001),#34852,
'DISTANCE_ACCURACY_VALUE',
'Maximum model space distance between geometric entities at asserted c
onnectivities');
#34817=(
GEOMETRIC_REPRESENTATION_CONTEXT(3)
GLOBAL_UNCERTAINTY_ASSIGNED_CONTEXT((#34763))
GLOBAL_UNIT_ASSIGNED_CONTEXT((#34852,#34854,#34855))
REPRESENTATION_CONTEXT('','3D')
);
#34851=(
GEOMETRIC_REPRESENTATION_CONTEXT(3)
GLOBAL_UNCERTAINTY_ASSIGNED_CONTEXT((#34797))
GLOBAL_UNIT_ASSIGNED_CONTEXT((#34852,#34854,#34855))
REPRESENTATION_CONTEXT('','3D')
);
#34852=(
LENGTH_UNIT()
NAMED_UNIT(*)
SI_UNIT(.CENTI.,.METRE.)
);
#34854=(
NAMED_UNIT(*)
PLANE_ANGLE_UNIT()
SI_UNIT($,.RADIAN.)
);
#34855=(
NAMED_UNIT(*)
SI_UNIT($,.STERADIAN.)
SOLID_ANGLE_UNIT()
);
#34875=SHAPE_DEFINITION_REPRESENTATION(#34928,#35092);
#34928=PRODUCT_DEFINITION_SHAPE('',$,#35146);
#35092=SHAPE_REPRESENTATION('',(#14709),#34817);
#35126=PRODUCT_DEFINITION_CONTEXT('part definition',#35287,'design');
#35146=PRODUCT_DEFINITION('Linear Guide Rail - 15 mm, 220 mm Long',
'Linear Guide Rail - 15 mm, 220 mm Long',#35199,#35126);
#35199=PRODUCT_DEFINITION_FORMATION('',$,#35308);
#35287=APPLICATION_CONTEXT(
'Core Data for Automotive Mechanical Design Process');
#35288=PRODUCT_CONTEXT('part definition',#35287,'mechanical');
#35308=PRODUCT('Linear Guide Rail - 15 mm, 220 mm Long',
'Linear Guide Rail - 15 mm, 220 mm Long',
'Linear Guide Rail - 15 mm, 220 mm Long',(#35288));
#35398=COLOUR_RGB('Sky Blue',0.24,0.69,0.87);
#35399=FILL_AREA_STYLE_COLOUR('',#35398);
#35400=FILL_AREA_STYLE('',(#35399));
#35401=SURFACE_STYLE_FILL_AREA(#35400);
#35402=SURFACE_SIDE_STYLE('',(#35401));
#35403=SURFACE_STYLE_USAGE(.BOTH.,#35402);
#35404=PRESENTATION_STYLE_ASSIGNMENT((#35403));
ENDSEC;
END-ISO-10303-21;
